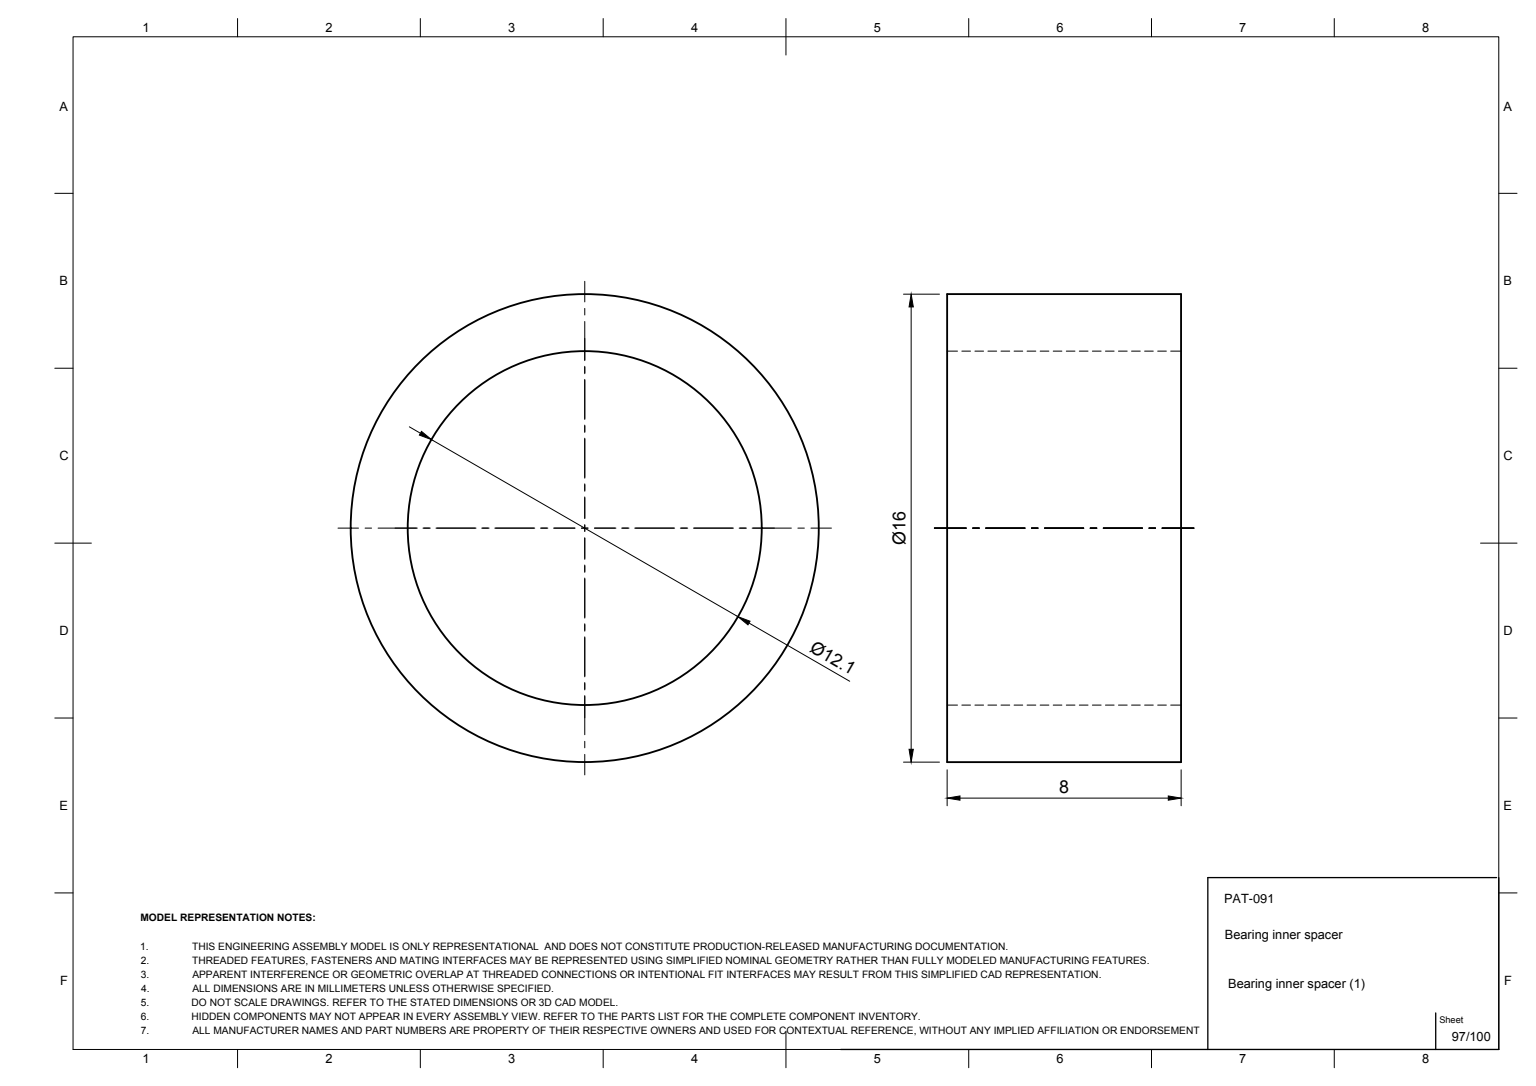
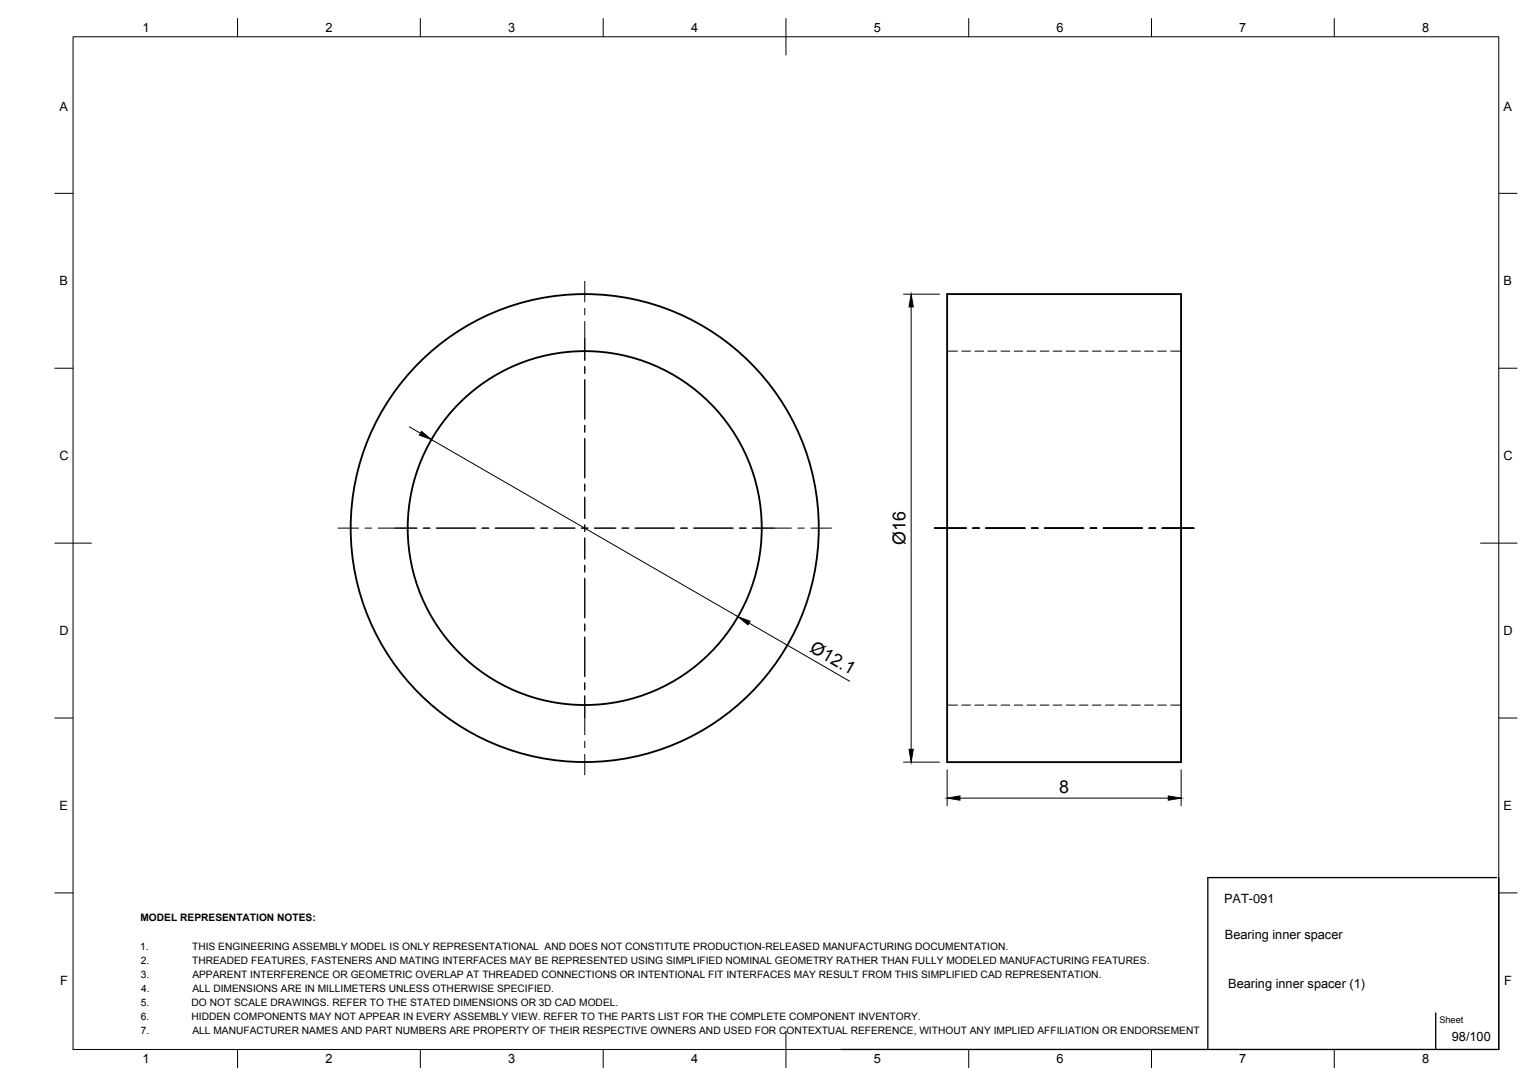
ISO-10303-21;
HEADER;
/* Generated by software containing ST-Developer
 * from STEP Tools, Inc. (www.steptools.com) 
 */

FILE_DESCRIPTION(
/* description */ ('PAT-091'),
/* implementation_level */ '2;1');

FILE_NAME(
/* name */ 'Bearing inner spacer.step',
/* time_stamp */ '2026-10-27T15:34:44-07:00',
/* author */ (''),
/* organization */ (''),
/* preprocessor_version */ 'ST-DEVELOPER v20.2',
/* originating_system */ 'Autodesk Translation Framework v15.17.0.0',
/* authorisation */ '');

FILE_SCHEMA (('AUTOMOTIVE_DESIGN { 1 0 10303 214 3 1 1 }'));
ENDSEC;

DATA;
#10=MECHANICAL_DESIGN_GEOMETRIC_PRESENTATION_REPRESENTATION('',(#1089),#25100);
#856=SHAPE_REPRESENTATION_RELATIONSHIP('SRR','None',#25625,#966);
#966=ADVANCED_BREP_SHAPE_REPRESENTATION('',(#1210),#25095);
#1089=STYLED_ITEM('',(#26191),#1210);
#1210=MANIFOLD_SOLID_BREP('Body1',#13369);
#1629=FACE_BOUND('',#4094,.T.);
#1630=FACE_BOUND('',#4096,.T.);
#2052=PLANE('',#16412);
#2053=PLANE('',#16413);
#2859=FACE_OUTER_BOUND('',#4091,.T.);
#2860=FACE_OUTER_BOUND('',#4092,.T.);
#2861=FACE_OUTER_BOUND('',#4093,.T.);
#2862=FACE_OUTER_BOUND('',#4095,.T.);
#4091=EDGE_LOOP('',(#12008,#12009,#12010,#12011));
#4092=EDGE_LOOP('',(#12012,#12013,#12014,#12015));
#4093=EDGE_LOOP('',(#12016));
#4094=EDGE_LOOP('',(#12017));
#4095=EDGE_LOOP('',(#12018));
#4096=EDGE_LOOP('',(#12019));
#4853=LINE('',#24768,#5593);
#4854=LINE('',#24774,#5594);
#5593=VECTOR('',#20843,0.605);
#5594=VECTOR('',#20850,0.8);
#6361=CIRCLE('',#16407,0.605);
#6362=CIRCLE('',#16408,0.605);
#6363=CIRCLE('',#16410,0.8);
#6364=CIRCLE('',#16411,0.8);
#7399=VERTEX_POINT('',#24765);
#7400=VERTEX_POINT('',#24767);
#7401=VERTEX_POINT('',#24771);
#7402=VERTEX_POINT('',#24773);
#8939=EDGE_CURVE('',#7399,#7399,#6361,.T.);
#8940=EDGE_CURVE('',#7399,#7400,#4853,.T.);
#8941=EDGE_CURVE('',#7400,#7400,#6362,.T.);
#8942=EDGE_CURVE('',#7401,#7401,#6363,.T.);
#8943=EDGE_CURVE('',#7401,#7402,#4854,.T.);
#8944=EDGE_CURVE('',#7402,#7402,#6364,.T.);
#12008=ORIENTED_EDGE('',*,*,#8939,.F.);
#12009=ORIENTED_EDGE('',*,*,#8940,.T.);
#12010=ORIENTED_EDGE('',*,*,#8941,.T.);
#12011=ORIENTED_EDGE('',*,*,#8940,.F.);
#12012=ORIENTED_EDGE('',*,*,#8942,.F.);
#12013=ORIENTED_EDGE('',*,*,#8943,.T.);
#12014=ORIENTED_EDGE('',*,*,#8944,.T.);
#12015=ORIENTED_EDGE('',*,*,#8943,.F.);
#12016=ORIENTED_EDGE('',*,*,#8942,.T.);
#12017=ORIENTED_EDGE('',*,*,#8939,.T.);
#12018=ORIENTED_EDGE('',*,*,#8944,.F.);
#12019=ORIENTED_EDGE('',*,*,#8941,.F.);
#12419=CYLINDRICAL_SURFACE('',#16406,0.605);
#12420=CYLINDRICAL_SURFACE('',#16409,0.8);
#13226=ADVANCED_FACE('',(#2859),#12419,.F.);
#13227=ADVANCED_FACE('',(#2860),#12420,.T.);
#13228=ADVANCED_FACE('',(#2861,#1629),#2052,.T.);
#13229=ADVANCED_FACE('',(#2862,#1630),#2053,.F.);
#13369=CLOSED_SHELL('',(#13226,#13227,#13228,#13229));
#16405=AXIS2_PLACEMENT_3D('',#24763,#20837,#20838);
#16406=AXIS2_PLACEMENT_3D('',#24764,#20839,#20840);
#16407=AXIS2_PLACEMENT_3D('',#24766,#20841,#20842);
#16408=AXIS2_PLACEMENT_3D('',#24769,#20844,#20845);
#16409=AXIS2_PLACEMENT_3D('',#24770,#20846,#20847);
#16410=AXIS2_PLACEMENT_3D('',#24772,#20848,#20849);
#16411=AXIS2_PLACEMENT_3D('',#24775,#20851,#20852);
#16412=AXIS2_PLACEMENT_3D('',#24776,#20853,#20854);
#16413=AXIS2_PLACEMENT_3D('',#24777,#20855,#20856);
#20837=DIRECTION('axis',(0.,0.,1.));
#20838=DIRECTION('refdir',(1.,0.,0.));
#20839=DIRECTION('center_axis',(1.,0.,0.));
#20840=DIRECTION('ref_axis',(0.,0.,-1.));
#20841=DIRECTION('center_axis',(-1.,0.,0.));
#20842=DIRECTION('ref_axis',(0.,0.,-1.));
#20843=DIRECTION('',(-1.,0.,0.));
#20844=DIRECTION('center_axis',(-1.,0.,0.));
#20845=DIRECTION('ref_axis',(0.,0.,-1.));
#20846=DIRECTION('center_axis',(1.,0.,0.));
#20847=DIRECTION('ref_axis',(0.,0.,-1.));
#20848=DIRECTION('center_axis',(1.,0.,0.));
#20849=DIRECTION('ref_axis',(0.,0.,-1.));
#20850=DIRECTION('',(-1.,0.,0.));
#20851=DIRECTION('center_axis',(1.,0.,0.));
#20852=DIRECTION('ref_axis',(0.,0.,-1.));
#20853=DIRECTION('center_axis',(1.,0.,0.));
#20854=DIRECTION('ref_axis',(0.,0.,-1.));
#20855=DIRECTION('center_axis',(1.,0.,0.));
#20856=DIRECTION('ref_axis',(0.,0.,-1.));
#24763=CARTESIAN_POINT('',(0.,0.,0.));
#24764=CARTESIAN_POINT('Origin',(-1.3,0.,6.));
#24765=CARTESIAN_POINT('',(-0.5,-7.40911313484149E-17,6.605));
#24766=CARTESIAN_POINT('Origin',(-0.5,0.,6.));
#24767=CARTESIAN_POINT('',(-1.3,-7.40911313484149E-17,6.605));
#24768=CARTESIAN_POINT('',(-1.3,-7.40911313484149E-17,6.605));
#24769=CARTESIAN_POINT('Origin',(-1.3,0.,6.));
#24770=CARTESIAN_POINT('Origin',(-1.3,0.,6.));
#24771=CARTESIAN_POINT('',(-0.5,-9.79717439317882E-17,6.8));
#24772=CARTESIAN_POINT('Origin',(-0.5,0.,6.));
#24773=CARTESIAN_POINT('',(-1.3,-9.79717439317882E-17,6.8));
#24774=CARTESIAN_POINT('',(-1.3,-9.79717439317882E-17,6.8));
#24775=CARTESIAN_POINT('Origin',(-1.3,0.,6.));
#24776=CARTESIAN_POINT('Origin',(-0.5,0.,6.));
#24777=CARTESIAN_POINT('Origin',(-1.3,0.,6.));
#24974=UNCERTAINTY_MEASURE_WITH_UNIT(LENGTH_MEASURE(0.001),#25101,
'DISTANCE_ACCURACY_VALUE',
'Maximum model space distance between geometric entities at asserted c
onnectivities');
#24979=UNCERTAINTY_MEASURE_WITH_UNIT(LENGTH_MEASURE(0.001),#25101,
'DISTANCE_ACCURACY_VALUE',
'Maximum model space distance between geometric entities at asserted c
onnectivities');
#25095=(
GEOMETRIC_REPRESENTATION_CONTEXT(3)
GLOBAL_UNCERTAINTY_ASSIGNED_CONTEXT((#24974))
GLOBAL_UNIT_ASSIGNED_CONTEXT((#25101,#25103,#25104))
REPRESENTATION_CONTEXT('','3D')
);
#25100=(
GEOMETRIC_REPRESENTATION_CONTEXT(3)
GLOBAL_UNCERTAINTY_ASSIGNED_CONTEXT((#24979))
GLOBAL_UNIT_ASSIGNED_CONTEXT((#25101,#25103,#25104))
REPRESENTATION_CONTEXT('','3D')
);
#25101=(
LENGTH_UNIT()
NAMED_UNIT(*)
SI_UNIT(.CENTI.,.METRE.)
);
#25103=(
NAMED_UNIT(*)
PLANE_ANGLE_UNIT()
SI_UNIT($,.RADIAN.)
);
#25104=(
NAMED_UNIT(*)
SI_UNIT($,.STERADIAN.)
SOLID_ANGLE_UNIT()
);
#25220=SHAPE_DEFINITION_REPRESENTATION(#25492,#25625);
#25492=PRODUCT_DEFINITION_SHAPE('',$,#25746);
#25625=SHAPE_REPRESENTATION('',(#16405),#25095);
#25630=PRODUCT_DEFINITION_CONTEXT('part definition',#25992,'design');
#25746=PRODUCT_DEFINITION('Bearing inner spacer','Bearing inner spacer',
#25866,#25630);
#25866=PRODUCT_DEFINITION_FORMATION('',$,#26109);
#25992=APPLICATION_CONTEXT(
'Core Data for Automotive Mechanical Design Process');
#25993=PRODUCT_CONTEXT('part definition',#25992,'mechanical');
#26109=PRODUCT('Bearing inner spacer','Bearing inner spacer',
'Bearing inner spacer',(#25993));
#26185=COLOUR_RGB('Grey',0.48,0.52,0.57);
#26186=FILL_AREA_STYLE_COLOUR('',#26185);
#26187=FILL_AREA_STYLE('',(#26186));
#26188=SURFACE_STYLE_FILL_AREA(#26187);
#26189=SURFACE_SIDE_STYLE('',(#26188));
#26190=SURFACE_STYLE_USAGE(.BOTH.,#26189);
#26191=PRESENTATION_STYLE_ASSIGNMENT((#26190));
ENDSEC;
END-ISO-10303-21;
